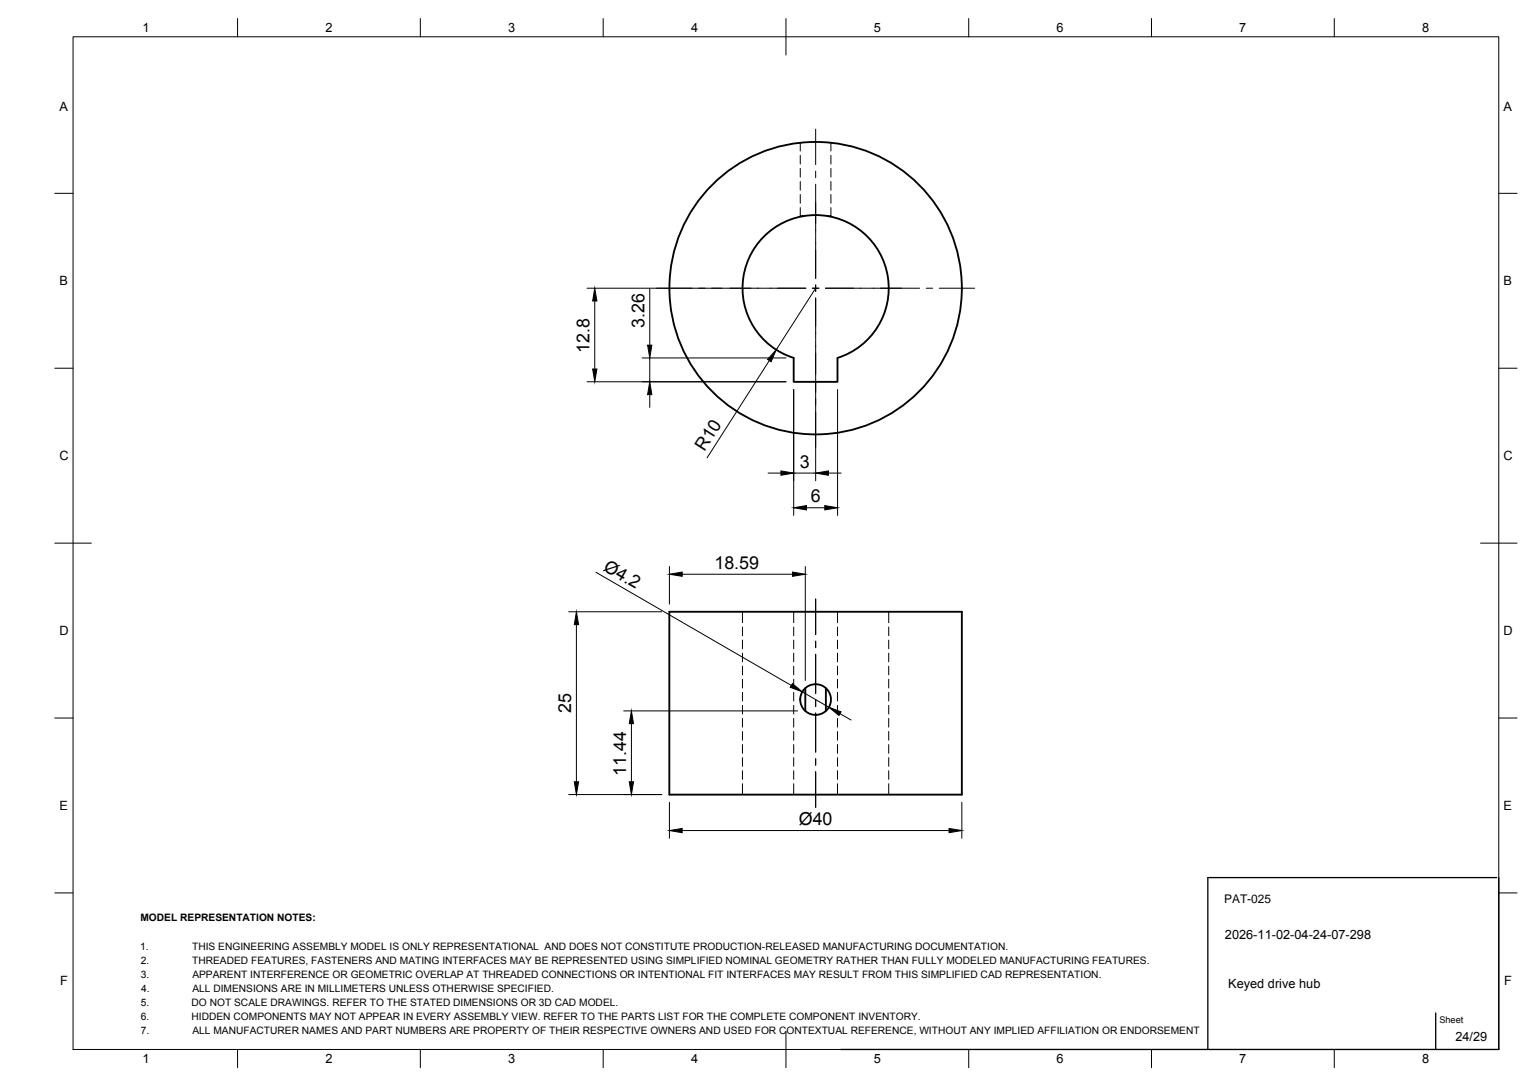
ISO-10303-21;
HEADER;
/* Generated by software containing ST-Developer
 * from STEP Tools, Inc. (www.steptools.com) 
 */

FILE_DESCRIPTION(
/* description */ ('Counter shaft with two pulleys and keyed hub'),
/* implementation_level */ '2;1');

FILE_NAME(
/* name */ 'Keyed drive hub.step',
/* time_stamp */ '2026-10-27T10:46:10-07:00',
/* author */ (''),
/* organization */ (''),
/* preprocessor_version */ 'ST-DEVELOPER v20.2',
/* originating_system */ 'Autodesk Translation Framework v15.17.0.0',
/* authorisation */ '');

FILE_SCHEMA (('AUTOMOTIVE_DESIGN { 1 0 10303 214 3 1 1 }'));
ENDSEC;

DATA;
#10=MECHANICAL_DESIGN_GEOMETRIC_PRESENTATION_REPRESENTATION('',(#308),#10821);
#208=B_SPLINE_CURVE_WITH_KNOTS('',3,(#9411,#9412,#9413,#9414,#9415,#9416,
#9417,#9418,#9419,#9420),.UNSPECIFIED.,.F.,.F.,(4,2,2,2,4),(0.803821788694082,
0.87295099185362,0.95230721290097,1.03166343394832,1.10079263710786),
 .UNSPECIFIED.);
#209=B_SPLINE_CURVE_WITH_KNOTS('',3,(#9426,#9427,#9428,#9429,#9430,#9431,
#9432,#9433,#9434,#9435,#9436,#9437,#9438,#9439,#9440,#9441,#9442,#9443),
 .UNSPECIFIED.,.F.,.F.,(4,2,2,2,2,2,2,2,4),(0.,0.0791670250779307,0.158334050155861,
0.237500747381213,0.316667444606564,0.395834141831916,0.475000839057267,
0.554167864135198,0.633334889213129),.UNSPECIFIED.);
#210=B_SPLINE_CURVE_WITH_KNOTS('',3,(#9444,#9445,#9446,#9447,#9448,#9449,
#9450,#9451,#9452,#9453,#9454,#9455,#9456,#9457,#9458,#9459,#9460,#9461),
 .UNSPECIFIED.,.F.,.F.,(4,2,2,2,2,2,2,2,4),(0.633334889213129,0.712501914291059,
0.79166893936899,0.870835636594341,0.950002333819693,1.02916903104504,1.1083357282704,
1.18750275334833,1.26666977842626),.UNSPECIFIED.);
#211=B_SPLINE_CURVE_WITH_KNOTS('',3,(#9464,#9465,#9466,#9467,#9468,#9469,
#9470,#9471,#9472,#9473),.UNSPECIFIED.,.F.,.F.,(4,2,2,2,4),(0.168950313426771,
0.238079516586307,0.317435737633657,0.396791958681006,0.465921161840543),
 .UNSPECIFIED.);
#257=SHAPE_REPRESENTATION_RELATIONSHIP('SRR','None',#10945,#282);
#282=ADVANCED_BREP_SHAPE_REPRESENTATION('',(#333),#10813);
#308=STYLED_ITEM('',(#11149),#333);
#333=MANIFOLD_SOLID_BREP('Body1',#5592);
#405=FACE_BOUND('',#1119,.T.);
#406=FACE_BOUND('',#1121,.T.);
#407=FACE_BOUND('',#1123,.T.);
#408=FACE_BOUND('',#1125,.T.);
#525=PLANE('',#6160);
#526=PLANE('',#6165);
#527=PLANE('',#6166);
#528=PLANE('',#6167);
#529=PLANE('',#6168);
#530=PLANE('',#6169);
#531=PLANE('',#6176);
#733=FACE_OUTER_BOUND('',#1112,.T.);
#734=FACE_OUTER_BOUND('',#1113,.T.);
#735=FACE_OUTER_BOUND('',#1114,.T.);
#736=FACE_OUTER_BOUND('',#1115,.T.);
#737=FACE_OUTER_BOUND('',#1116,.T.);
#738=FACE_OUTER_BOUND('',#1117,.T.);
#739=FACE_OUTER_BOUND('',#1118,.T.);
#740=FACE_OUTER_BOUND('',#1120,.T.);
#741=FACE_OUTER_BOUND('',#1122,.T.);
#742=FACE_OUTER_BOUND('',#1124,.T.);
#1112=EDGE_LOOP('',(#4219,#4220));
#1113=EDGE_LOOP('',(#4221,#4222,#4223,#4224,#4225,#4226,#4227,#4228,#4229));
#1114=EDGE_LOOP('',(#4230,#4231,#4232));
#1115=EDGE_LOOP('',(#4233,#4234,#4235,#4236));
#1116=EDGE_LOOP('',(#4237,#4238,#4239,#4240));
#1117=EDGE_LOOP('',(#4241,#4242,#4243,#4244));
#1118=EDGE_LOOP('',(#4245));
#1119=EDGE_LOOP('',(#4246,#4247,#4248,#4249));
#1120=EDGE_LOOP('',(#4250,#4251,#4252,#4253));
#1121=EDGE_LOOP('',(#4254,#4255,#4256,#4257));
#1122=EDGE_LOOP('',(#4258,#4259,#4260,#4261));
#1123=EDGE_LOOP('',(#4262,#4263));
#1124=EDGE_LOOP('',(#4264));
#1125=EDGE_LOOP('',(#4265,#4266,#4267,#4268));
#1481=LINE('',#9407,#1870);
#1482=LINE('',#9424,#1871);
#1483=LINE('',#9475,#1872);
#1484=LINE('',#9479,#1873);
#1485=LINE('',#9481,#1874);
#1486=LINE('',#9483,#1875);
#1487=LINE('',#9484,#1876);
#1488=LINE('',#9487,#1877);
#1489=LINE('',#9489,#1878);
#1490=LINE('',#9490,#1879);
#1491=LINE('',#9493,#1880);
#1492=LINE('',#9495,#1881);
#1493=LINE('',#9496,#1882);
#1494=LINE('',#9505,#1883);
#1870=VECTOR('',#7301,1.);
#1871=VECTOR('',#7308,0.21);
#1872=VECTOR('',#7313,1.);
#1873=VECTOR('',#7316,1.);
#1874=VECTOR('',#7317,1.);
#1875=VECTOR('',#7318,1.);
#1876=VECTOR('',#7319,1.);
#1877=VECTOR('',#7322,1.);
#1878=VECTOR('',#7323,1.);
#1879=VECTOR('',#7324,1.);
#1880=VECTOR('',#7327,1.);
#1881=VECTOR('',#7328,1.);
#1882=VECTOR('',#7329,1.);
#1883=VECTOR('',#7342,2.);
#2182=CIRCLE('',#6161,0.21);
#2183=CIRCLE('',#6163,0.21);
#2184=CIRCLE('',#6164,0.21);
#2185=CIRCLE('',#6170,2.);
#2186=CIRCLE('',#6171,1.);
#2187=CIRCLE('',#6173,1.);
#2188=CIRCLE('',#6175,2.);
#2587=VERTEX_POINT('',#9405);
#2588=VERTEX_POINT('',#9406);
#2589=VERTEX_POINT('',#9410);
#2590=VERTEX_POINT('',#9421);
#2591=VERTEX_POINT('',#9423);
#2592=VERTEX_POINT('',#9425);
#2593=VERTEX_POINT('',#9462);
#2594=VERTEX_POINT('',#9477);
#2595=VERTEX_POINT('',#9478);
#2596=VERTEX_POINT('',#9480);
#2597=VERTEX_POINT('',#9482);
#2598=VERTEX_POINT('',#9486);
#2599=VERTEX_POINT('',#9488);
#2600=VERTEX_POINT('',#9492);
#2601=VERTEX_POINT('',#9494);
#2602=VERTEX_POINT('',#9498);
#2603=VERTEX_POINT('',#9504);
#3182=EDGE_CURVE('',#2587,#2588,#1481,.T.);
#3183=EDGE_CURVE('',#2587,#2588,#2182,.T.);
#3184=EDGE_CURVE('',#2589,#2587,#208,.T.);
#3185=EDGE_CURVE('',#2590,#2589,#2183,.T.);
#3186=EDGE_CURVE('',#2590,#2591,#1482,.T.);
#3187=EDGE_CURVE('',#2592,#2591,#209,.T.);
#3188=EDGE_CURVE('',#2591,#2592,#210,.T.);
#3189=EDGE_CURVE('',#2593,#2590,#2184,.T.);
#3190=EDGE_CURVE('',#2588,#2593,#211,.T.);
#3191=EDGE_CURVE('',#2593,#2589,#1483,.T.);
#3192=EDGE_CURVE('',#2594,#2595,#1484,.T.);
#3193=EDGE_CURVE('',#2594,#2596,#1485,.T.);
#3194=EDGE_CURVE('',#2597,#2596,#1486,.T.);
#3195=EDGE_CURVE('',#2595,#2597,#1487,.T.);
#3196=EDGE_CURVE('',#2598,#2594,#1488,.T.);
#3197=EDGE_CURVE('',#2598,#2599,#1489,.T.);
#3198=EDGE_CURVE('',#2596,#2599,#1490,.T.);
#3199=EDGE_CURVE('',#2600,#2598,#1491,.T.);
#3200=EDGE_CURVE('',#2601,#2600,#1492,.T.);
#3201=EDGE_CURVE('',#2599,#2601,#1493,.T.);
#3202=EDGE_CURVE('',#2602,#2602,#2185,.T.);
#3203=EDGE_CURVE('',#2601,#2597,#2186,.T.);
#3204=EDGE_CURVE('',#2600,#2595,#2187,.T.);
#3205=EDGE_CURVE('',#2602,#2603,#1494,.T.);
#3206=EDGE_CURVE('',#2603,#2603,#2188,.T.);
#4219=ORIENTED_EDGE('',*,*,#3182,.F.);
#4220=ORIENTED_EDGE('',*,*,#3183,.T.);
#4221=ORIENTED_EDGE('',*,*,#3184,.F.);
#4222=ORIENTED_EDGE('',*,*,#3185,.F.);
#4223=ORIENTED_EDGE('',*,*,#3186,.T.);
#4224=ORIENTED_EDGE('',*,*,#3187,.F.);
#4225=ORIENTED_EDGE('',*,*,#3188,.F.);
#4226=ORIENTED_EDGE('',*,*,#3186,.F.);
#4227=ORIENTED_EDGE('',*,*,#3189,.F.);
#4228=ORIENTED_EDGE('',*,*,#3190,.F.);
#4229=ORIENTED_EDGE('',*,*,#3183,.F.);
#4230=ORIENTED_EDGE('',*,*,#3191,.F.);
#4231=ORIENTED_EDGE('',*,*,#3189,.T.);
#4232=ORIENTED_EDGE('',*,*,#3185,.T.);
#4233=ORIENTED_EDGE('',*,*,#3192,.F.);
#4234=ORIENTED_EDGE('',*,*,#3193,.T.);
#4235=ORIENTED_EDGE('',*,*,#3194,.F.);
#4236=ORIENTED_EDGE('',*,*,#3195,.F.);
#4237=ORIENTED_EDGE('',*,*,#3196,.F.);
#4238=ORIENTED_EDGE('',*,*,#3197,.T.);
#4239=ORIENTED_EDGE('',*,*,#3198,.F.);
#4240=ORIENTED_EDGE('',*,*,#3193,.F.);
#4241=ORIENTED_EDGE('',*,*,#3199,.F.);
#4242=ORIENTED_EDGE('',*,*,#3200,.F.);
#4243=ORIENTED_EDGE('',*,*,#3201,.F.);
#4244=ORIENTED_EDGE('',*,*,#3197,.F.);
#4245=ORIENTED_EDGE('',*,*,#3202,.T.);
#4246=ORIENTED_EDGE('',*,*,#3194,.T.);
#4247=ORIENTED_EDGE('',*,*,#3198,.T.);
#4248=ORIENTED_EDGE('',*,*,#3201,.T.);
#4249=ORIENTED_EDGE('',*,*,#3203,.T.);
#4250=ORIENTED_EDGE('',*,*,#3195,.T.);
#4251=ORIENTED_EDGE('',*,*,#3203,.F.);
#4252=ORIENTED_EDGE('',*,*,#3200,.T.);
#4253=ORIENTED_EDGE('',*,*,#3204,.T.);
#4254=ORIENTED_EDGE('',*,*,#3190,.T.);
#4255=ORIENTED_EDGE('',*,*,#3191,.T.);
#4256=ORIENTED_EDGE('',*,*,#3184,.T.);
#4257=ORIENTED_EDGE('',*,*,#3182,.T.);
#4258=ORIENTED_EDGE('',*,*,#3202,.F.);
#4259=ORIENTED_EDGE('',*,*,#3205,.T.);
#4260=ORIENTED_EDGE('',*,*,#3206,.T.);
#4261=ORIENTED_EDGE('',*,*,#3205,.F.);
#4262=ORIENTED_EDGE('',*,*,#3187,.T.);
#4263=ORIENTED_EDGE('',*,*,#3188,.T.);
#4264=ORIENTED_EDGE('',*,*,#3206,.F.);
#4265=ORIENTED_EDGE('',*,*,#3192,.T.);
#4266=ORIENTED_EDGE('',*,*,#3204,.F.);
#4267=ORIENTED_EDGE('',*,*,#3199,.T.);
#4268=ORIENTED_EDGE('',*,*,#3196,.T.);
#5159=CYLINDRICAL_SURFACE('',#6162,0.21);
#5160=CYLINDRICAL_SURFACE('',#6172,1.);
#5161=CYLINDRICAL_SURFACE('',#6174,2.);
#5404=ADVANCED_FACE('',(#733),#525,.T.);
#5405=ADVANCED_FACE('',(#734),#5159,.F.);
#5406=ADVANCED_FACE('',(#735),#526,.T.);
#5407=ADVANCED_FACE('',(#736),#527,.F.);
#5408=ADVANCED_FACE('',(#737),#528,.F.);
#5409=ADVANCED_FACE('',(#738),#529,.F.);
#5410=ADVANCED_FACE('',(#739,#405),#530,.T.);
#5411=ADVANCED_FACE('',(#740,#406),#5160,.F.);
#5412=ADVANCED_FACE('',(#741,#407),#5161,.T.);
#5413=ADVANCED_FACE('',(#742,#408),#531,.F.);
#5592=CLOSED_SHELL('',(#5404,#5405,#5406,#5407,#5408,#5409,#5410,#5411,
#5412,#5413));
#6159=AXIS2_PLACEMENT_3D('',#9403,#7297,#7298);
#6160=AXIS2_PLACEMENT_3D('',#9404,#7299,#7300);
#6161=AXIS2_PLACEMENT_3D('',#9408,#7302,#7303);
#6162=AXIS2_PLACEMENT_3D('',#9409,#7304,#7305);
#6163=AXIS2_PLACEMENT_3D('',#9422,#7306,#7307);
#6164=AXIS2_PLACEMENT_3D('',#9463,#7309,#7310);
#6165=AXIS2_PLACEMENT_3D('',#9474,#7311,#7312);
#6166=AXIS2_PLACEMENT_3D('',#9476,#7314,#7315);
#6167=AXIS2_PLACEMENT_3D('',#9485,#7320,#7321);
#6168=AXIS2_PLACEMENT_3D('',#9491,#7325,#7326);
#6169=AXIS2_PLACEMENT_3D('',#9497,#7330,#7331);
#6170=AXIS2_PLACEMENT_3D('',#9499,#7332,#7333);
#6171=AXIS2_PLACEMENT_3D('',#9500,#7334,#7335);
#6172=AXIS2_PLACEMENT_3D('',#9501,#7336,#7337);
#6173=AXIS2_PLACEMENT_3D('',#9502,#7338,#7339);
#6174=AXIS2_PLACEMENT_3D('',#9503,#7340,#7341);
#6175=AXIS2_PLACEMENT_3D('',#9506,#7343,#7344);
#6176=AXIS2_PLACEMENT_3D('',#9507,#7345,#7346);
#7297=DIRECTION('axis',(0.,0.,1.));
#7298=DIRECTION('refdir',(1.,0.,0.));
#7299=DIRECTION('center_axis',(0.,0.,1.));
#7300=DIRECTION('ref_axis',(1.,0.,0.));
#7301=DIRECTION('',(0.,1.,0.));
#7302=DIRECTION('center_axis',(0.,0.,1.));
#7303=DIRECTION('ref_axis',(1.,0.,0.));
#7304=DIRECTION('center_axis',(0.,0.,1.));
#7305=DIRECTION('ref_axis',(1.,0.,0.));
#7306=DIRECTION('center_axis',(0.,0.,1.));
#7307=DIRECTION('ref_axis',(1.,0.,0.));
#7308=DIRECTION('',(0.,0.,1.));
#7309=DIRECTION('center_axis',(0.,0.,1.));
#7310=DIRECTION('ref_axis',(1.,0.,0.));
#7311=DIRECTION('center_axis',(0.,0.,1.));
#7312=DIRECTION('ref_axis',(1.,0.,0.));
#7313=DIRECTION('',(0.,-1.,0.));
#7314=DIRECTION('center_axis',(-1.,0.,0.));
#7315=DIRECTION('ref_axis',(0.,0.,1.));
#7316=DIRECTION('',(0.,0.,1.));
#7317=DIRECTION('',(0.,1.,0.));
#7318=DIRECTION('',(0.,0.,-1.));
#7319=DIRECTION('',(0.,1.,0.));
#7320=DIRECTION('center_axis',(0.,0.,-1.));
#7321=DIRECTION('ref_axis',(-1.,0.,0.));
#7322=DIRECTION('',(-1.,0.,0.));
#7323=DIRECTION('',(0.,1.,0.));
#7324=DIRECTION('',(1.,0.,0.));
#7325=DIRECTION('center_axis',(1.,0.,0.));
#7326=DIRECTION('ref_axis',(0.,0.,-1.));
#7327=DIRECTION('',(0.,0.,-1.));
#7328=DIRECTION('',(0.,-1.,0.));
#7329=DIRECTION('',(0.,0.,1.));
#7330=DIRECTION('center_axis',(0.,1.,0.));
#7331=DIRECTION('ref_axis',(1.,0.,0.));
#7332=DIRECTION('center_axis',(0.,1.,0.));
#7333=DIRECTION('ref_axis',(1.,0.,0.));
#7334=DIRECTION('center_axis',(0.,-1.,0.));
#7335=DIRECTION('ref_axis',(1.,0.,0.));
#7336=DIRECTION('center_axis',(0.,1.,0.));
#7337=DIRECTION('ref_axis',(-1.83697019872103E-16,0.,1.));
#7338=DIRECTION('center_axis',(0.,-1.,0.));
#7339=DIRECTION('ref_axis',(1.,0.,0.));
#7340=DIRECTION('center_axis',(0.,1.,0.));
#7341=DIRECTION('ref_axis',(1.,0.,0.));
#7342=DIRECTION('',(0.,-1.,0.));
#7343=DIRECTION('center_axis',(0.,1.,0.));
#7344=DIRECTION('ref_axis',(1.,0.,0.));
#7345=DIRECTION('center_axis',(0.,1.,0.));
#7346=DIRECTION('ref_axis',(1.,0.,0.));
#9403=CARTESIAN_POINT('',(0.,0.,0.));
#9404=CARTESIAN_POINT('Origin',(0.,10.2,5.52));
#9405=CARTESIAN_POINT('',(0.141067359796651,10.044436508139,5.52));
#9406=CARTESIAN_POINT('',(0.141067359796651,10.355563491861,5.52));
#9407=CARTESIAN_POINT('',(0.141067359796651,9.,5.52));
#9408=CARTESIAN_POINT('Origin',(0.,10.2,5.52));
#9409=CARTESIAN_POINT('Origin',(0.,10.2,5.52));
#9410=CARTESIAN_POINT('',(-0.141067359796651,10.044436508139,5.52));
#9411=CARTESIAN_POINT('Ctrl Pts',(-0.141067359796651,10.044436508139,5.52));
#9412=CARTESIAN_POINT('Ctrl Pts',(-0.123818356698219,10.0287948476368,5.52245784982447));
#9413=CARTESIAN_POINT('Ctrl Pts',(-0.102998643109696,10.015375956669,5.52493819304946));
#9414=CARTESIAN_POINT('Ctrl Pts',(-0.0546141143983528,9.99530253627557,
5.52884449237241));
#9415=CARTESIAN_POINT('Ctrl Pts',(-0.0264520736824499,9.99,5.53));
#9416=CARTESIAN_POINT('Ctrl Pts',(0.0264520736824499,9.99,5.53));
#9417=CARTESIAN_POINT('Ctrl Pts',(0.0546141143983523,9.99530253627557,5.52884449237241));
#9418=CARTESIAN_POINT('Ctrl Pts',(0.102998643109696,10.015375956669,5.52493819304946));
#9419=CARTESIAN_POINT('Ctrl Pts',(0.123818356698219,10.0287948476368,5.52245784982447));
#9420=CARTESIAN_POINT('Ctrl Pts',(0.141067359796652,10.044436508139,5.52));
#9421=CARTESIAN_POINT('',(-0.21,10.2,5.52));
#9422=CARTESIAN_POINT('Origin',(0.,10.2,5.52));
#9423=CARTESIAN_POINT('',(-0.21,10.2,6.51894444366855));
#9424=CARTESIAN_POINT('',(-0.21,10.2,5.52));
#9425=CARTESIAN_POINT('',(0.21,10.2,6.51894444366855));
#9426=CARTESIAN_POINT('Ctrl Pts',(0.21,10.2,6.51894444366855));
#9427=CARTESIAN_POINT('Ctrl Pts',(0.21,10.1736109916407,6.51894444366855));
#9428=CARTESIAN_POINT('Ctrl Pts',(0.204722164681422,10.1454764062218,6.51952376620524));
#9429=CARTESIAN_POINT('Ctrl Pts',(0.183284867450471,10.0937425531788,6.52161307432363));
#9430=CARTESIAN_POINT('Ctrl Pts',(0.167126466290584,10.0701416181922,6.52309254589373));
#9431=CARTESIAN_POINT('Ctrl Pts',(0.129858458976496,10.0328736108781,6.52586721250997));
#9432=CARTESIAN_POINT('Ctrl Pts',(0.106257490219277,10.0167151494345,6.527343117591));
#9433=CARTESIAN_POINT('Ctrl Pts',(0.0545235237847863,9.99527780741314,6.52942425936951));
#9434=CARTESIAN_POINT('Ctrl Pts',(0.0263888990751172,9.99,6.53));
#9435=CARTESIAN_POINT('Ctrl Pts',(-0.0263888990751171,9.99,6.53));
#9436=CARTESIAN_POINT('Ctrl Pts',(-0.0545235237847855,9.99527780741314,
6.52942425936951));
#9437=CARTESIAN_POINT('Ctrl Pts',(-0.106257490219277,10.0167151494345,6.527343117591));
#9438=CARTESIAN_POINT('Ctrl Pts',(-0.129858458976496,10.0328736108781,6.52586721250997));
#9439=CARTESIAN_POINT('Ctrl Pts',(-0.167126466290584,10.0701416181922,6.52309254589373));
#9440=CARTESIAN_POINT('Ctrl Pts',(-0.183284867450472,10.0937425531788,6.52161307432363));
#9441=CARTESIAN_POINT('Ctrl Pts',(-0.204722164681422,10.1454764062218,6.51952376620524));
#9442=CARTESIAN_POINT('Ctrl Pts',(-0.21,10.1736109916407,6.51894444366855));
#9443=CARTESIAN_POINT('Ctrl Pts',(-0.21,10.2,6.51894444366855));
#9444=CARTESIAN_POINT('Ctrl Pts',(-0.21,10.2,6.51894444366855));
#9445=CARTESIAN_POINT('Ctrl Pts',(-0.21,10.2263890083593,6.51894444366855));
#9446=CARTESIAN_POINT('Ctrl Pts',(-0.204722164681422,10.2545235937782,6.51952376620524));
#9447=CARTESIAN_POINT('Ctrl Pts',(-0.183284867450471,10.3062574468212,6.52161307432363));
#9448=CARTESIAN_POINT('Ctrl Pts',(-0.167126466290584,10.3298583818078,6.52309254589373));
#9449=CARTESIAN_POINT('Ctrl Pts',(-0.129858458976496,10.3671263891219,6.52586721250997));
#9450=CARTESIAN_POINT('Ctrl Pts',(-0.106257490219277,10.3832848505655,6.527343117591));
#9451=CARTESIAN_POINT('Ctrl Pts',(-0.0545235237847863,10.4047221925869,
6.52942425936951));
#9452=CARTESIAN_POINT('Ctrl Pts',(-0.0263888990751172,10.41,6.53));
#9453=CARTESIAN_POINT('Ctrl Pts',(0.0263888990751171,10.41,6.53));
#9454=CARTESIAN_POINT('Ctrl Pts',(0.0545235237847861,10.4047221925869,6.52942425936951));
#9455=CARTESIAN_POINT('Ctrl Pts',(0.106257490219277,10.3832848505655,6.527343117591));
#9456=CARTESIAN_POINT('Ctrl Pts',(0.129858458976496,10.3671263891219,6.52586721250997));
#9457=CARTESIAN_POINT('Ctrl Pts',(0.167126466290584,10.3298583818078,6.52309254589373));
#9458=CARTESIAN_POINT('Ctrl Pts',(0.183284867450471,10.3062574468212,6.52161307432363));
#9459=CARTESIAN_POINT('Ctrl Pts',(0.204722164681422,10.2545235937782,6.51952376620524));
#9460=CARTESIAN_POINT('Ctrl Pts',(0.21,10.2263890083593,6.51894444366855));
#9461=CARTESIAN_POINT('Ctrl Pts',(0.21,10.2,6.51894444366855));
#9462=CARTESIAN_POINT('',(-0.141067359796651,10.355563491861,5.52));
#9463=CARTESIAN_POINT('Origin',(0.,10.2,5.52));
#9464=CARTESIAN_POINT('Ctrl Pts',(0.14106735979665,10.355563491861,5.52));
#9465=CARTESIAN_POINT('Ctrl Pts',(0.123818356698217,10.3712051523632,5.52245784982447));
#9466=CARTESIAN_POINT('Ctrl Pts',(0.102998643109696,10.384624043331,5.52493819304946));
#9467=CARTESIAN_POINT('Ctrl Pts',(0.0546141143983528,10.4046974637244,5.52884449237241));
#9468=CARTESIAN_POINT('Ctrl Pts',(0.0264520736824499,10.41,5.53));
#9469=CARTESIAN_POINT('Ctrl Pts',(-0.0264520736824498,10.41,5.53));
#9470=CARTESIAN_POINT('Ctrl Pts',(-0.0546141143983515,10.4046974637244,
5.52884449237241));
#9471=CARTESIAN_POINT('Ctrl Pts',(-0.102998643109696,10.384624043331,5.52493819304946));
#9472=CARTESIAN_POINT('Ctrl Pts',(-0.123818356698217,10.3712051523632,5.52245784982447));
#9473=CARTESIAN_POINT('Ctrl Pts',(-0.14106735979665,10.355563491861,5.52));
#9474=CARTESIAN_POINT('Origin',(0.,10.2,5.52));
#9475=CARTESIAN_POINT('',(-0.141067359796651,9.,5.52));
#9476=CARTESIAN_POINT('Origin',(-0.3,8.9,3.25));
#9477=CARTESIAN_POINT('',(-0.3,9.,3.25));
#9478=CARTESIAN_POINT('',(-0.3,9.,3.57606079858305));
#9479=CARTESIAN_POINT('',(-0.3,9.,3.89));
#9480=CARTESIAN_POINT('',(-0.3,11.5,3.25));
#9481=CARTESIAN_POINT('',(-0.3,8.9,3.25));
#9482=CARTESIAN_POINT('',(-0.3,11.5,3.57606079858305));
#9483=CARTESIAN_POINT('',(-0.3,11.5,3.89));
#9484=CARTESIAN_POINT('',(-0.3,9.,3.57606079858305));
#9485=CARTESIAN_POINT('Origin',(0.3,8.9,3.25));
#9486=CARTESIAN_POINT('',(0.3,9.,3.25));
#9487=CARTESIAN_POINT('',(0.15,9.,3.25));
#9488=CARTESIAN_POINT('',(0.3,11.5,3.25));
#9489=CARTESIAN_POINT('',(0.3,8.9,3.25));
#9490=CARTESIAN_POINT('',(0.15,11.5,3.25));
#9491=CARTESIAN_POINT('Origin',(0.3,8.9,4.53));
#9492=CARTESIAN_POINT('',(0.3,9.,3.57606079858305));
#9493=CARTESIAN_POINT('',(0.3,9.,4.53));
#9494=CARTESIAN_POINT('',(0.3,11.5,3.57606079858305));
#9495=CARTESIAN_POINT('',(0.3,9.,3.57606079858305));
#9496=CARTESIAN_POINT('',(0.3,11.5,4.53));
#9497=CARTESIAN_POINT('Origin',(0.,11.5,4.53));
#9498=CARTESIAN_POINT('',(-2.,11.5,4.53));
#9499=CARTESIAN_POINT('Origin',(0.,11.5,4.53));
#9500=CARTESIAN_POINT('Origin',(0.,11.5,4.53));
#9501=CARTESIAN_POINT('Origin',(0.,9.,4.53));
#9502=CARTESIAN_POINT('Origin',(0.,9.,4.53));
#9503=CARTESIAN_POINT('Origin',(0.,9.,4.53));
#9504=CARTESIAN_POINT('',(-2.,9.,4.53));
#9505=CARTESIAN_POINT('',(-2.,9.,4.53));
#9506=CARTESIAN_POINT('Origin',(0.,9.,4.53));
#9507=CARTESIAN_POINT('Origin',(0.,9.,4.53));
#10783=UNCERTAINTY_MEASURE_WITH_UNIT(LENGTH_MEASURE(0.001),#10822,
'DISTANCE_ACCURACY_VALUE',
'Maximum model space distance between geometric entities at asserted c
onnectivities');
#10791=UNCERTAINTY_MEASURE_WITH_UNIT(LENGTH_MEASURE(0.001),#10822,
'DISTANCE_ACCURACY_VALUE',
'Maximum model space distance between geometric entities at asserted c
onnectivities');
#10813=(
GEOMETRIC_REPRESENTATION_CONTEXT(3)
GLOBAL_UNCERTAINTY_ASSIGNED_CONTEXT((#10783))
GLOBAL_UNIT_ASSIGNED_CONTEXT((#10822,#10824,#10825))
REPRESENTATION_CONTEXT('','3D')
);
#10821=(
GEOMETRIC_REPRESENTATION_CONTEXT(3)
GLOBAL_UNCERTAINTY_ASSIGNED_CONTEXT((#10791))
GLOBAL_UNIT_ASSIGNED_CONTEXT((#10822,#10824,#10825))
REPRESENTATION_CONTEXT('','3D')
);
#10822=(
LENGTH_UNIT()
NAMED_UNIT(*)
SI_UNIT(.CENTI.,.METRE.)
);
#10824=(
NAMED_UNIT(*)
PLANE_ANGLE_UNIT()
SI_UNIT($,.RADIAN.)
);
#10825=(
NAMED_UNIT(*)
SI_UNIT($,.STERADIAN.)
SOLID_ANGLE_UNIT()
);
#10847=SHAPE_DEFINITION_REPRESENTATION(#10895,#10945);
#10895=PRODUCT_DEFINITION_SHAPE('',$,#10975);
#10945=SHAPE_REPRESENTATION('',(#6159),#10813);
#10953=PRODUCT_DEFINITION_CONTEXT('part definition',#11042,'design');
#10975=PRODUCT_DEFINITION('Keyed drive hub','Keyed drive hub',#11004,#10953);
#11004=PRODUCT_DEFINITION_FORMATION('',$,#11065);
#11042=APPLICATION_CONTEXT(
'Core Data for Automotive Mechanical Design Process');
#11043=PRODUCT_CONTEXT('part definition',#11042,'mechanical');
#11065=PRODUCT('Keyed drive hub','Keyed drive hub','Keyed drive hub',(#11043));
#11143=COLOUR_RGB('Off White',0.89,0.88,0.83);
#11144=FILL_AREA_STYLE_COLOUR('',#11143);
#11145=FILL_AREA_STYLE('',(#11144));
#11146=SURFACE_STYLE_FILL_AREA(#11145);
#11147=SURFACE_SIDE_STYLE('',(#11146));
#11148=SURFACE_STYLE_USAGE(.BOTH.,#11147);
#11149=PRESENTATION_STYLE_ASSIGNMENT((#11148));
ENDSEC;
END-ISO-10303-21;
